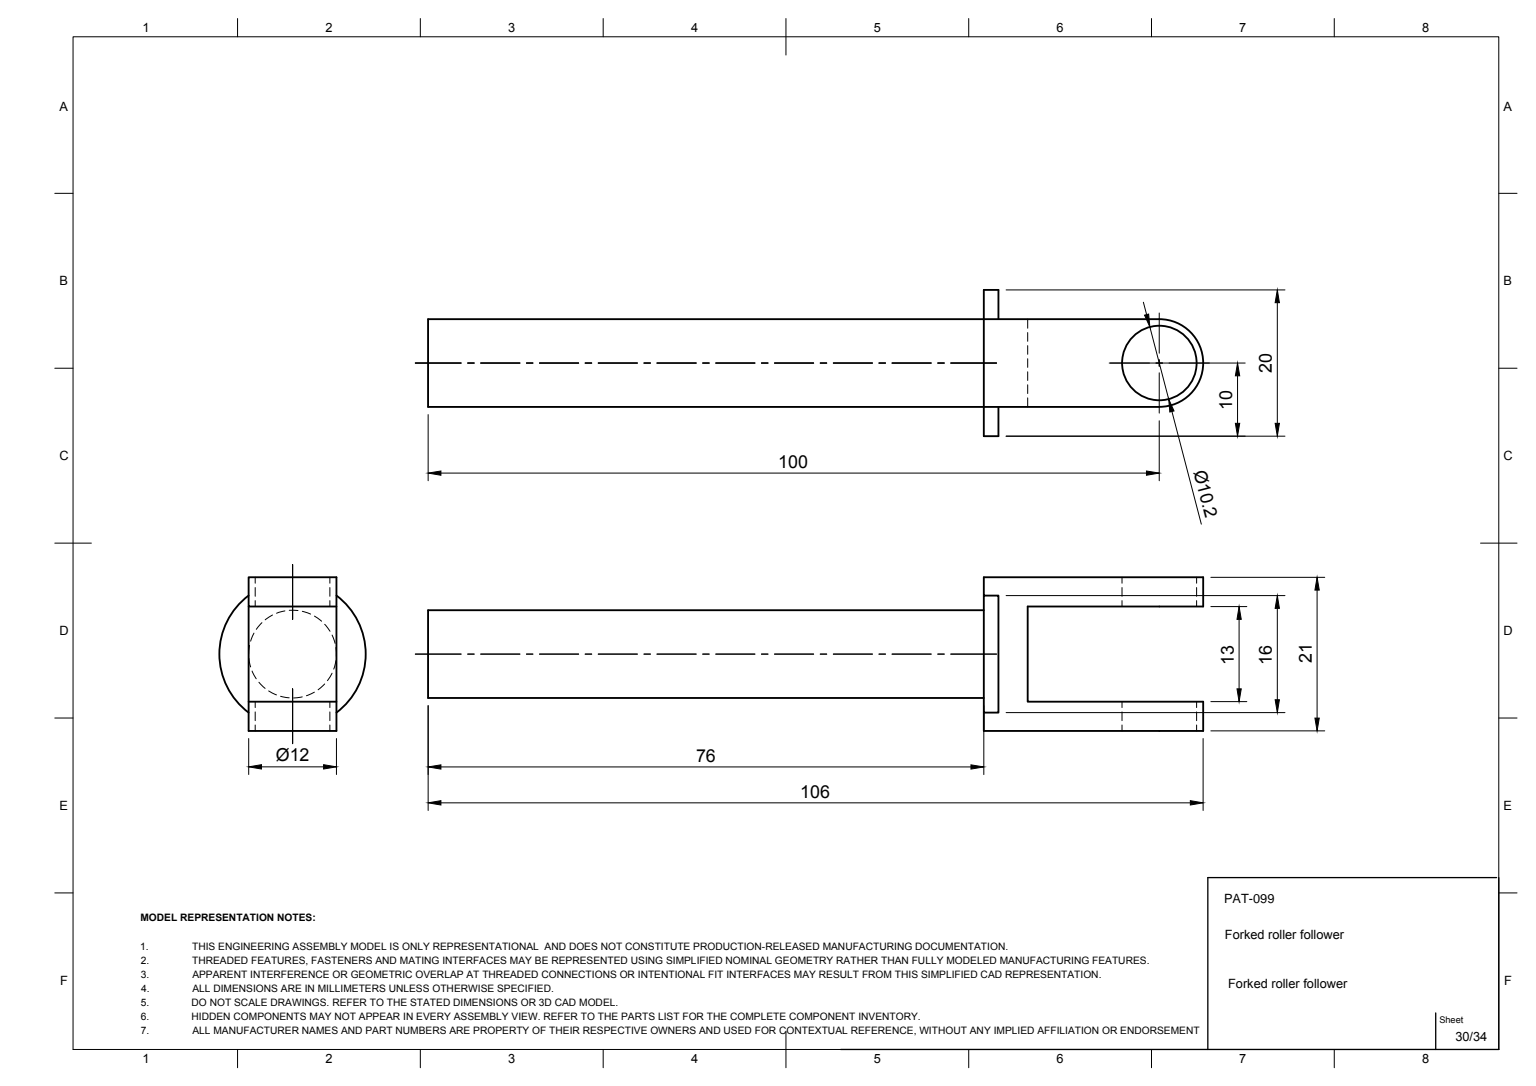
ISO-10303-21;
HEADER;
/* Generated by software containing ST-Developer
 * from STEP Tools, Inc. (www.steptools.com) 
 */

FILE_DESCRIPTION(
/* description */ ('PAT-099'),
/* implementation_level */ '2;1');

FILE_NAME(
/* name */ 'Forked roller follower.step',
/* time_stamp */ '2026-10-29T17:25:42-07:00',
/* author */ (''),
/* organization */ (''),
/* preprocessor_version */ 'ST-DEVELOPER v20.2',
/* originating_system */ 'Autodesk Translation Framework v15.17.0.0',
/* authorisation */ '');

FILE_SCHEMA (('AUTOMOTIVE_DESIGN { 1 0 10303 214 3 1 1 }'));
ENDSEC;

DATA;
#10=MECHANICAL_DESIGN_GEOMETRIC_PRESENTATION_REPRESENTATION('',(#351),#11035);
#301=SHAPE_REPRESENTATION_RELATIONSHIP('SRR','None',#11172,#326);
#326=ADVANCED_BREP_SHAPE_REPRESENTATION('',(#383),#11022);
#351=STYLED_ITEM('',(#11400),#383);
#383=MANIFOLD_SOLID_BREP('Body1',#4720);
#500=FACE_BOUND('',#1221,.T.);
#501=FACE_BOUND('',#1227,.T.);
#502=FACE_BOUND('',#1229,.T.);
#503=FACE_BOUND('',#1233,.T.);
#504=FACE_BOUND('',#1235,.T.);
#610=PLANE('',#5398);
#611=PLANE('',#5400);
#612=PLANE('',#5406);
#613=PLANE('',#5408);
#614=PLANE('',#5418);
#615=PLANE('',#5419);
#616=PLANE('',#5420);
#617=PLANE('',#5424);
#618=PLANE('',#5425);
#619=PLANE('',#5428);
#620=PLANE('',#5429);
#836=FACE_OUTER_BOUND('',#1216,.T.);
#837=FACE_OUTER_BOUND('',#1217,.T.);
#838=FACE_OUTER_BOUND('',#1218,.T.);
#839=FACE_OUTER_BOUND('',#1219,.T.);
#840=FACE_OUTER_BOUND('',#1220,.T.);
#841=FACE_OUTER_BOUND('',#1222,.T.);
#842=FACE_OUTER_BOUND('',#1223,.T.);
#843=FACE_OUTER_BOUND('',#1224,.T.);
#844=FACE_OUTER_BOUND('',#1225,.T.);
#845=FACE_OUTER_BOUND('',#1226,.T.);
#846=FACE_OUTER_BOUND('',#1228,.T.);
#847=FACE_OUTER_BOUND('',#1230,.T.);
#848=FACE_OUTER_BOUND('',#1231,.T.);
#849=FACE_OUTER_BOUND('',#1232,.T.);
#850=FACE_OUTER_BOUND('',#1234,.T.);
#851=FACE_OUTER_BOUND('',#1236,.T.);
#852=FACE_OUTER_BOUND('',#1237,.T.);
#853=FACE_OUTER_BOUND('',#1238,.T.);
#1216=EDGE_LOOP('',(#3893,#3894));
#1217=EDGE_LOOP('',(#3895,#3896));
#1218=EDGE_LOOP('',(#3897,#3898,#3899,#3900));
#1219=EDGE_LOOP('',(#3901,#3902,#3903,#3904));
#1220=EDGE_LOOP('',(#3905,#3906,#3907,#3908,#3909,#3910,#3911,#3912));
#1221=EDGE_LOOP('',(#3913));
#1222=EDGE_LOOP('',(#3914,#3915,#3916,#3917,#3918,#3919,#3920,#3921,#3922,
#3923,#3924,#3925));
#1223=EDGE_LOOP('',(#3926,#3927,#3928,#3929));
#1224=EDGE_LOOP('',(#3930,#3931,#3932,#3933));
#1225=EDGE_LOOP('',(#3934,#3935,#3936,#3937));
#1226=EDGE_LOOP('',(#3938,#3939,#3940,#3941));
#1227=EDGE_LOOP('',(#3942));
#1228=EDGE_LOOP('',(#3943,#3944,#3945,#3946));
#1229=EDGE_LOOP('',(#3947));
#1230=EDGE_LOOP('',(#3948,#3949,#3950,#3951,#3952,#3953,#3954,#3955,#3956,
#3957,#3958,#3959));
#1231=EDGE_LOOP('',(#3960,#3961,#3962,#3963));
#1232=EDGE_LOOP('',(#3964,#3965,#3966,#3967));
#1233=EDGE_LOOP('',(#3968));
#1234=EDGE_LOOP('',(#3969,#3970,#3971,#3972));
#1235=EDGE_LOOP('',(#3973));
#1236=EDGE_LOOP('',(#3974,#3975,#3976,#3977));
#1237=EDGE_LOOP('',(#3978));
#1238=EDGE_LOOP('',(#3979,#3980,#3981,#3982));
#1516=LINE('',#10121,#1768);
#1517=LINE('',#10126,#1769);
#1518=LINE('',#10130,#1770);
#1519=LINE('',#10133,#1771);
#1520=LINE('',#10136,#1772);
#1521=LINE('',#10138,#1773);
#1522=LINE('',#10142,#1774);
#1523=LINE('',#10144,#1775);
#1524=LINE('',#10145,#1776);
#1525=LINE('',#10147,#1777);
#1526=LINE('',#10149,#1778);
#1527=LINE('',#10150,#1779);
#1528=LINE('',#10155,#1780);
#1529=LINE('',#10157,#1781);
#1530=LINE('',#10159,#1782);
#1531=LINE('',#10161,#1783);
#1532=LINE('',#10163,#1784);
#1533=LINE('',#10165,#1785);
#1534=LINE('',#10166,#1786);
#1535=LINE('',#10171,#1787);
#1536=LINE('',#10177,#1788);
#1537=LINE('',#10182,#1789);
#1538=LINE('',#10186,#1790);
#1539=LINE('',#10189,#1791);
#1540=LINE('',#10190,#1792);
#1541=LINE('',#10193,#1793);
#1542=LINE('',#10195,#1794);
#1543=LINE('',#10197,#1795);
#1544=LINE('',#10198,#1796);
#1545=LINE('',#10204,#1797);
#1546=LINE('',#10208,#1798);
#1768=VECTOR('',#6607,1.);
#1769=VECTOR('',#6612,1.);
#1770=VECTOR('',#6617,1.);
#1771=VECTOR('',#6620,1.);
#1772=VECTOR('',#6623,1.);
#1773=VECTOR('',#6624,1.);
#1774=VECTOR('',#6629,1.);
#1775=VECTOR('',#6630,1.);
#1776=VECTOR('',#6631,1.);
#1777=VECTOR('',#6632,1.);
#1778=VECTOR('',#6633,1.);
#1779=VECTOR('',#6634,1.);
#1780=VECTOR('',#6639,1.);
#1781=VECTOR('',#6640,1.);
#1782=VECTOR('',#6641,1.);
#1783=VECTOR('',#6642,1.);
#1784=VECTOR('',#6643,1.);
#1785=VECTOR('',#6644,1.);
#1786=VECTOR('',#6645,1.);
#1787=VECTOR('',#6650,0.51);
#1788=VECTOR('',#6657,0.51);
#1789=VECTOR('',#6662,1.);
#1790=VECTOR('',#6669,1.);
#1791=VECTOR('',#6672,1.);
#1792=VECTOR('',#6673,1.);
#1793=VECTOR('',#6676,1.);
#1794=VECTOR('',#6677,1.);
#1795=VECTOR('',#6678,1.);
#1796=VECTOR('',#6679,1.);
#1797=VECTOR('',#6690,1.);
#1798=VECTOR('',#6695,0.6);
#2027=CIRCLE('',#5399,1.);
#2028=CIRCLE('',#5401,1.);
#2029=CIRCLE('',#5403,1.);
#2030=CIRCLE('',#5405,1.);
#2031=CIRCLE('',#5407,0.6);
#2032=CIRCLE('',#5410,0.51);
#2033=CIRCLE('',#5411,0.51);
#2034=CIRCLE('',#5413,0.51);
#2035=CIRCLE('',#5414,0.51);
#2036=CIRCLE('',#5416,0.6);
#2037=CIRCLE('',#5417,0.6);
#2038=CIRCLE('',#5422,0.6);
#2039=CIRCLE('',#5423,0.6);
#2040=CIRCLE('',#5427,0.6);
#2395=VERTEX_POINT('',#10119);
#2396=VERTEX_POINT('',#10120);
#2397=VERTEX_POINT('',#10124);
#2398=VERTEX_POINT('',#10125);
#2399=VERTEX_POINT('',#10129);
#2400=VERTEX_POINT('',#10131);
#2401=VERTEX_POINT('',#10135);
#2402=VERTEX_POINT('',#10137);
#2403=VERTEX_POINT('',#10141);
#2404=VERTEX_POINT('',#10143);
#2405=VERTEX_POINT('',#10146);
#2406=VERTEX_POINT('',#10148);
#2407=VERTEX_POINT('',#10151);
#2408=VERTEX_POINT('',#10154);
#2409=VERTEX_POINT('',#10156);
#2410=VERTEX_POINT('',#10158);
#2411=VERTEX_POINT('',#10160);
#2412=VERTEX_POINT('',#10162);
#2413=VERTEX_POINT('',#10164);
#2414=VERTEX_POINT('',#10168);
#2415=VERTEX_POINT('',#10170);
#2416=VERTEX_POINT('',#10174);
#2417=VERTEX_POINT('',#10176);
#2418=VERTEX_POINT('',#10180);
#2419=VERTEX_POINT('',#10181);
#2420=VERTEX_POINT('',#10188);
#2421=VERTEX_POINT('',#10192);
#2422=VERTEX_POINT('',#10194);
#2423=VERTEX_POINT('',#10196);
#2424=VERTEX_POINT('',#10206);
#2923=EDGE_CURVE('',#2395,#2396,#1516,.T.);
#2924=EDGE_CURVE('',#2396,#2395,#2027,.T.);
#2925=EDGE_CURVE('',#2397,#2398,#1517,.T.);
#2926=EDGE_CURVE('',#2398,#2397,#2028,.T.);
#2927=EDGE_CURVE('',#2399,#2395,#1518,.T.);
#2928=EDGE_CURVE('',#2400,#2399,#2029,.T.);
#2929=EDGE_CURVE('',#2396,#2400,#1519,.T.);
#2930=EDGE_CURVE('',#2398,#2401,#1520,.T.);
#2931=EDGE_CURVE('',#2402,#2397,#1521,.T.);
#2932=EDGE_CURVE('',#2401,#2402,#2030,.T.);
#2933=EDGE_CURVE('',#2402,#2403,#1522,.T.);
#2934=EDGE_CURVE('',#2403,#2404,#1523,.T.);
#2935=EDGE_CURVE('',#2404,#2400,#1524,.T.);
#2936=EDGE_CURVE('',#2399,#2405,#1525,.T.);
#2937=EDGE_CURVE('',#2405,#2406,#1526,.T.);
#2938=EDGE_CURVE('',#2406,#2401,#1527,.T.);
#2939=EDGE_CURVE('',#2407,#2407,#2031,.T.);
#2940=EDGE_CURVE('',#2408,#2404,#1528,.T.);
#2941=EDGE_CURVE('',#2409,#2408,#1529,.T.);
#2942=EDGE_CURVE('',#2409,#2410,#1530,.T.);
#2943=EDGE_CURVE('',#2410,#2411,#1531,.T.);
#2944=EDGE_CURVE('',#2412,#2411,#1532,.T.);
#2945=EDGE_CURVE('',#2413,#2412,#1533,.T.);
#2946=EDGE_CURVE('',#2413,#2405,#1534,.T.);
#2947=EDGE_CURVE('',#2414,#2414,#2032,.T.);
#2948=EDGE_CURVE('',#2414,#2415,#1535,.T.);
#2949=EDGE_CURVE('',#2415,#2415,#2033,.T.);
#2950=EDGE_CURVE('',#2416,#2416,#2034,.T.);
#2951=EDGE_CURVE('',#2416,#2417,#1536,.T.);
#2952=EDGE_CURVE('',#2417,#2417,#2035,.T.);
#2953=EDGE_CURVE('',#2418,#2419,#1537,.T.);
#2954=EDGE_CURVE('',#2418,#2409,#2036,.T.);
#2955=EDGE_CURVE('',#2419,#2408,#2037,.T.);
#2956=EDGE_CURVE('',#2419,#2403,#1538,.T.);
#2957=EDGE_CURVE('',#2420,#2418,#1539,.T.);
#2958=EDGE_CURVE('',#2410,#2420,#1540,.T.);
#2959=EDGE_CURVE('',#2421,#2406,#1541,.T.);
#2960=EDGE_CURVE('',#2421,#2422,#1542,.T.);
#2961=EDGE_CURVE('',#2423,#2422,#1543,.T.);
#2962=EDGE_CURVE('',#2423,#2420,#1544,.T.);
#2963=EDGE_CURVE('',#2422,#2412,#2038,.T.);
#2964=EDGE_CURVE('',#2421,#2413,#2039,.T.);
#2965=EDGE_CURVE('',#2423,#2411,#1545,.T.);
#2966=EDGE_CURVE('',#2424,#2424,#2040,.T.);
#2967=EDGE_CURVE('',#2424,#2407,#1546,.T.);
#3893=ORIENTED_EDGE('',*,*,#2923,.F.);
#3894=ORIENTED_EDGE('',*,*,#2924,.F.);
#3895=ORIENTED_EDGE('',*,*,#2925,.F.);
#3896=ORIENTED_EDGE('',*,*,#2926,.F.);
#3897=ORIENTED_EDGE('',*,*,#2927,.F.);
#3898=ORIENTED_EDGE('',*,*,#2928,.F.);
#3899=ORIENTED_EDGE('',*,*,#2929,.F.);
#3900=ORIENTED_EDGE('',*,*,#2924,.T.);
#3901=ORIENTED_EDGE('',*,*,#2930,.F.);
#3902=ORIENTED_EDGE('',*,*,#2926,.T.);
#3903=ORIENTED_EDGE('',*,*,#2931,.F.);
#3904=ORIENTED_EDGE('',*,*,#2932,.F.);
#3905=ORIENTED_EDGE('',*,*,#2933,.T.);
#3906=ORIENTED_EDGE('',*,*,#2934,.T.);
#3907=ORIENTED_EDGE('',*,*,#2935,.T.);
#3908=ORIENTED_EDGE('',*,*,#2928,.T.);
#3909=ORIENTED_EDGE('',*,*,#2936,.T.);
#3910=ORIENTED_EDGE('',*,*,#2937,.T.);
#3911=ORIENTED_EDGE('',*,*,#2938,.T.);
#3912=ORIENTED_EDGE('',*,*,#2932,.T.);
#3913=ORIENTED_EDGE('',*,*,#2939,.F.);
#3914=ORIENTED_EDGE('',*,*,#2927,.T.);
#3915=ORIENTED_EDGE('',*,*,#2923,.T.);
#3916=ORIENTED_EDGE('',*,*,#2929,.T.);
#3917=ORIENTED_EDGE('',*,*,#2935,.F.);
#3918=ORIENTED_EDGE('',*,*,#2940,.F.);
#3919=ORIENTED_EDGE('',*,*,#2941,.F.);
#3920=ORIENTED_EDGE('',*,*,#2942,.T.);
#3921=ORIENTED_EDGE('',*,*,#2943,.T.);
#3922=ORIENTED_EDGE('',*,*,#2944,.F.);
#3923=ORIENTED_EDGE('',*,*,#2945,.F.);
#3924=ORIENTED_EDGE('',*,*,#2946,.T.);
#3925=ORIENTED_EDGE('',*,*,#2936,.F.);
#3926=ORIENTED_EDGE('',*,*,#2947,.F.);
#3927=ORIENTED_EDGE('',*,*,#2948,.T.);
#3928=ORIENTED_EDGE('',*,*,#2949,.F.);
#3929=ORIENTED_EDGE('',*,*,#2948,.F.);
#3930=ORIENTED_EDGE('',*,*,#2950,.F.);
#3931=ORIENTED_EDGE('',*,*,#2951,.T.);
#3932=ORIENTED_EDGE('',*,*,#2952,.F.);
#3933=ORIENTED_EDGE('',*,*,#2951,.F.);
#3934=ORIENTED_EDGE('',*,*,#2953,.F.);
#3935=ORIENTED_EDGE('',*,*,#2954,.T.);
#3936=ORIENTED_EDGE('',*,*,#2941,.T.);
#3937=ORIENTED_EDGE('',*,*,#2955,.F.);
#3938=ORIENTED_EDGE('',*,*,#2940,.T.);
#3939=ORIENTED_EDGE('',*,*,#2934,.F.);
#3940=ORIENTED_EDGE('',*,*,#2956,.F.);
#3941=ORIENTED_EDGE('',*,*,#2955,.T.);
#3942=ORIENTED_EDGE('',*,*,#2952,.T.);
#3943=ORIENTED_EDGE('',*,*,#2957,.F.);
#3944=ORIENTED_EDGE('',*,*,#2958,.F.);
#3945=ORIENTED_EDGE('',*,*,#2942,.F.);
#3946=ORIENTED_EDGE('',*,*,#2954,.F.);
#3947=ORIENTED_EDGE('',*,*,#2950,.T.);
#3948=ORIENTED_EDGE('',*,*,#2930,.T.);
#3949=ORIENTED_EDGE('',*,*,#2938,.F.);
#3950=ORIENTED_EDGE('',*,*,#2959,.F.);
#3951=ORIENTED_EDGE('',*,*,#2960,.T.);
#3952=ORIENTED_EDGE('',*,*,#2961,.F.);
#3953=ORIENTED_EDGE('',*,*,#2962,.T.);
#3954=ORIENTED_EDGE('',*,*,#2957,.T.);
#3955=ORIENTED_EDGE('',*,*,#2953,.T.);
#3956=ORIENTED_EDGE('',*,*,#2956,.T.);
#3957=ORIENTED_EDGE('',*,*,#2933,.F.);
#3958=ORIENTED_EDGE('',*,*,#2931,.T.);
#3959=ORIENTED_EDGE('',*,*,#2925,.T.);
#3960=ORIENTED_EDGE('',*,*,#2945,.T.);
#3961=ORIENTED_EDGE('',*,*,#2963,.F.);
#3962=ORIENTED_EDGE('',*,*,#2960,.F.);
#3963=ORIENTED_EDGE('',*,*,#2964,.T.);
#3964=ORIENTED_EDGE('',*,*,#2959,.T.);
#3965=ORIENTED_EDGE('',*,*,#2937,.F.);
#3966=ORIENTED_EDGE('',*,*,#2946,.F.);
#3967=ORIENTED_EDGE('',*,*,#2964,.F.);
#3968=ORIENTED_EDGE('',*,*,#2947,.T.);
#3969=ORIENTED_EDGE('',*,*,#2944,.T.);
#3970=ORIENTED_EDGE('',*,*,#2965,.F.);
#3971=ORIENTED_EDGE('',*,*,#2961,.T.);
#3972=ORIENTED_EDGE('',*,*,#2963,.T.);
#3973=ORIENTED_EDGE('',*,*,#2949,.T.);
#3974=ORIENTED_EDGE('',*,*,#2966,.F.);
#3975=ORIENTED_EDGE('',*,*,#2967,.T.);
#3976=ORIENTED_EDGE('',*,*,#2939,.T.);
#3977=ORIENTED_EDGE('',*,*,#2967,.F.);
#3978=ORIENTED_EDGE('',*,*,#2966,.T.);
#3979=ORIENTED_EDGE('',*,*,#2958,.T.);
#3980=ORIENTED_EDGE('',*,*,#2962,.F.);
#3981=ORIENTED_EDGE('',*,*,#2965,.T.);
#3982=ORIENTED_EDGE('',*,*,#2943,.F.);
#4394=CYLINDRICAL_SURFACE('',#5402,1.);
#4395=CYLINDRICAL_SURFACE('',#5404,1.);
#4396=CYLINDRICAL_SURFACE('',#5409,0.51);
#4397=CYLINDRICAL_SURFACE('',#5412,0.51);
#4398=CYLINDRICAL_SURFACE('',#5415,0.6);
#4399=CYLINDRICAL_SURFACE('',#5421,0.6);
#4400=CYLINDRICAL_SURFACE('',#5426,0.6);
#4601=ADVANCED_FACE('',(#836),#610,.F.);
#4602=ADVANCED_FACE('',(#837),#611,.F.);
#4603=ADVANCED_FACE('',(#838),#4394,.T.);
#4604=ADVANCED_FACE('',(#839),#4395,.T.);
#4605=ADVANCED_FACE('',(#840,#500),#612,.T.);
#4606=ADVANCED_FACE('',(#841),#613,.T.);
#4607=ADVANCED_FACE('',(#842),#4396,.F.);
#4608=ADVANCED_FACE('',(#843),#4397,.F.);
#4609=ADVANCED_FACE('',(#844),#4398,.T.);
#4610=ADVANCED_FACE('',(#845,#501),#614,.T.);
#4611=ADVANCED_FACE('',(#846,#502),#615,.F.);
#4612=ADVANCED_FACE('',(#847),#616,.T.);
#4613=ADVANCED_FACE('',(#848),#4399,.T.);
#4614=ADVANCED_FACE('',(#849,#503),#617,.T.);
#4615=ADVANCED_FACE('',(#850,#504),#618,.T.);
#4616=ADVANCED_FACE('',(#851),#4400,.T.);
#4617=ADVANCED_FACE('',(#852),#619,.T.);
#4618=ADVANCED_FACE('',(#853),#620,.F.);
#4720=CLOSED_SHELL('',(#4601,#4602,#4603,#4604,#4605,#4606,#4607,#4608,
#4609,#4610,#4611,#4612,#4613,#4614,#4615,#4616,#4617,#4618));
#5397=AXIS2_PLACEMENT_3D('',#10117,#6603,#6604);
#5398=AXIS2_PLACEMENT_3D('',#10118,#6605,#6606);
#5399=AXIS2_PLACEMENT_3D('',#10122,#6608,#6609);
#5400=AXIS2_PLACEMENT_3D('',#10123,#6610,#6611);
#5401=AXIS2_PLACEMENT_3D('',#10127,#6613,#6614);
#5402=AXIS2_PLACEMENT_3D('',#10128,#6615,#6616);
#5403=AXIS2_PLACEMENT_3D('',#10132,#6618,#6619);
#5404=AXIS2_PLACEMENT_3D('',#10134,#6621,#6622);
#5405=AXIS2_PLACEMENT_3D('',#10139,#6625,#6626);
#5406=AXIS2_PLACEMENT_3D('',#10140,#6627,#6628);
#5407=AXIS2_PLACEMENT_3D('',#10152,#6635,#6636);
#5408=AXIS2_PLACEMENT_3D('',#10153,#6637,#6638);
#5409=AXIS2_PLACEMENT_3D('',#10167,#6646,#6647);
#5410=AXIS2_PLACEMENT_3D('',#10169,#6648,#6649);
#5411=AXIS2_PLACEMENT_3D('',#10172,#6651,#6652);
#5412=AXIS2_PLACEMENT_3D('',#10173,#6653,#6654);
#5413=AXIS2_PLACEMENT_3D('',#10175,#6655,#6656);
#5414=AXIS2_PLACEMENT_3D('',#10178,#6658,#6659);
#5415=AXIS2_PLACEMENT_3D('',#10179,#6660,#6661);
#5416=AXIS2_PLACEMENT_3D('',#10183,#6663,#6664);
#5417=AXIS2_PLACEMENT_3D('',#10184,#6665,#6666);
#5418=AXIS2_PLACEMENT_3D('',#10185,#6667,#6668);
#5419=AXIS2_PLACEMENT_3D('',#10187,#6670,#6671);
#5420=AXIS2_PLACEMENT_3D('',#10191,#6674,#6675);
#5421=AXIS2_PLACEMENT_3D('',#10199,#6680,#6681);
#5422=AXIS2_PLACEMENT_3D('',#10200,#6682,#6683);
#5423=AXIS2_PLACEMENT_3D('',#10201,#6684,#6685);
#5424=AXIS2_PLACEMENT_3D('',#10202,#6686,#6687);
#5425=AXIS2_PLACEMENT_3D('',#10203,#6688,#6689);
#5426=AXIS2_PLACEMENT_3D('',#10205,#6691,#6692);
#5427=AXIS2_PLACEMENT_3D('',#10207,#6693,#6694);
#5428=AXIS2_PLACEMENT_3D('',#10209,#6696,#6697);
#5429=AXIS2_PLACEMENT_3D('',#10210,#6698,#6699);
#6603=DIRECTION('axis',(0.,0.,1.));
#6604=DIRECTION('refdir',(1.,0.,0.));
#6605=DIRECTION('center_axis',(1.,0.,0.));
#6606=DIRECTION('ref_axis',(0.,0.,-1.));
#6607=DIRECTION('',(0.,0.,1.));
#6608=DIRECTION('center_axis',(1.,0.,0.));
#6609=DIRECTION('ref_axis',(0.,0.,-1.));
#6610=DIRECTION('center_axis',(1.,0.,0.));
#6611=DIRECTION('ref_axis',(0.,0.,-1.));
#6612=DIRECTION('',(0.,0.,-1.));
#6613=DIRECTION('center_axis',(1.,0.,0.));
#6614=DIRECTION('ref_axis',(0.,0.,-1.));
#6615=DIRECTION('center_axis',(1.,0.,0.));
#6616=DIRECTION('ref_axis',(0.,0.,-1.));
#6617=DIRECTION('',(-1.,0.,0.));
#6618=DIRECTION('center_axis',(1.,0.,0.));
#6619=DIRECTION('ref_axis',(0.,0.,-1.));
#6620=DIRECTION('',(1.,0.,0.));
#6621=DIRECTION('center_axis',(1.,0.,0.));
#6622=DIRECTION('ref_axis',(0.,0.,-1.));
#6623=DIRECTION('',(1.,0.,0.));
#6624=DIRECTION('',(-1.,0.,0.));
#6625=DIRECTION('center_axis',(1.,0.,0.));
#6626=DIRECTION('ref_axis',(0.,0.,-1.));
#6627=DIRECTION('center_axis',(1.,0.,0.));
#6628=DIRECTION('ref_axis',(0.,0.,-1.));
#6629=DIRECTION('',(0.,0.,1.));
#6630=DIRECTION('',(0.,-1.,0.));
#6631=DIRECTION('',(0.,0.,-1.));
#6632=DIRECTION('',(0.,0.,-1.));
#6633=DIRECTION('',(0.,1.,0.));
#6634=DIRECTION('',(0.,0.,1.));
#6635=DIRECTION('center_axis',(1.,0.,0.));
#6636=DIRECTION('ref_axis',(0.,0.,-1.));
#6637=DIRECTION('center_axis',(0.,-1.,0.));
#6638=DIRECTION('ref_axis',(0.,0.,-1.));
#6639=DIRECTION('',(1.,0.,0.));
#6640=DIRECTION('',(0.,0.,1.));
#6641=DIRECTION('',(1.,0.,0.));
#6642=DIRECTION('',(0.,0.,-1.));
#6643=DIRECTION('',(1.,0.,0.));
#6644=DIRECTION('',(0.,0.,1.));
#6645=DIRECTION('',(1.,0.,0.));
#6646=DIRECTION('center_axis',(0.,0.,1.));
#6647=DIRECTION('ref_axis',(1.,0.,0.));
#6648=DIRECTION('center_axis',(0.,0.,1.));
#6649=DIRECTION('ref_axis',(1.,0.,0.));
#6650=DIRECTION('',(0.,0.,1.));
#6651=DIRECTION('center_axis',(0.,0.,-1.));
#6652=DIRECTION('ref_axis',(1.,0.,0.));
#6653=DIRECTION('center_axis',(0.,0.,1.));
#6654=DIRECTION('ref_axis',(1.,0.,0.));
#6655=DIRECTION('center_axis',(0.,0.,1.));
#6656=DIRECTION('ref_axis',(1.,0.,0.));
#6657=DIRECTION('',(0.,0.,1.));
#6658=DIRECTION('center_axis',(0.,0.,-1.));
#6659=DIRECTION('ref_axis',(1.,0.,0.));
#6660=DIRECTION('center_axis',(0.,0.,1.));
#6661=DIRECTION('ref_axis',(-1.,1.22464679914735E-16,0.));
#6662=DIRECTION('',(0.,0.,1.));
#6663=DIRECTION('center_axis',(0.,0.,1.));
#6664=DIRECTION('ref_axis',(1.,0.,0.));
#6665=DIRECTION('center_axis',(0.,0.,1.));
#6666=DIRECTION('ref_axis',(1.,0.,0.));
#6667=DIRECTION('center_axis',(0.,0.,1.));
#6668=DIRECTION('ref_axis',(0.,-1.,0.));
#6669=DIRECTION('',(1.,0.,0.));
#6670=DIRECTION('center_axis',(0.,0.,1.));
#6671=DIRECTION('ref_axis',(1.,0.,0.));
#6672=DIRECTION('',(-1.,0.,0.));
#6673=DIRECTION('',(0.,1.,0.));
#6674=DIRECTION('center_axis',(0.,1.,0.));
#6675=DIRECTION('ref_axis',(0.,0.,1.));
#6676=DIRECTION('',(1.,0.,0.));
#6677=DIRECTION('',(0.,0.,1.));
#6678=DIRECTION('',(-1.,0.,0.));
#6679=DIRECTION('',(0.,0.,1.));
#6680=DIRECTION('center_axis',(0.,0.,1.));
#6681=DIRECTION('ref_axis',(-1.,-1.22464679914735E-16,0.));
#6682=DIRECTION('center_axis',(0.,0.,1.));
#6683=DIRECTION('ref_axis',(1.,0.,0.));
#6684=DIRECTION('center_axis',(0.,0.,1.));
#6685=DIRECTION('ref_axis',(1.,0.,0.));
#6686=DIRECTION('center_axis',(0.,0.,-1.));
#6687=DIRECTION('ref_axis',(0.,1.,0.));
#6688=DIRECTION('center_axis',(0.,0.,1.));
#6689=DIRECTION('ref_axis',(1.,0.,0.));
#6690=DIRECTION('',(0.,-1.,0.));
#6691=DIRECTION('center_axis',(1.,0.,0.));
#6692=DIRECTION('ref_axis',(0.,0.,-1.));
#6693=DIRECTION('center_axis',(1.,0.,0.));
#6694=DIRECTION('ref_axis',(0.,0.,-1.));
#6695=DIRECTION('',(-1.,0.,0.));
#6696=DIRECTION('center_axis',(1.,0.,0.));
#6697=DIRECTION('ref_axis',(0.,0.,-1.));
#6698=DIRECTION('center_axis',(1.,0.,0.));
#6699=DIRECTION('ref_axis',(0.,0.,-1.));
#10117=CARTESIAN_POINT('',(0.,0.,0.));
#10118=CARTESIAN_POINT('Origin',(6.2,0.,5.25));
#10119=CARTESIAN_POINT('',(6.2,-0.6,4.45));
#10120=CARTESIAN_POINT('',(6.2,-0.6,6.05));
#10121=CARTESIAN_POINT('',(6.2,-0.6,5.775));
#10122=CARTESIAN_POINT('Origin',(6.2,0.,5.25));
#10123=CARTESIAN_POINT('Origin',(6.2,0.,5.25));
#10124=CARTESIAN_POINT('',(6.2,0.6,6.05));
#10125=CARTESIAN_POINT('',(6.2,0.6,4.45));
#10126=CARTESIAN_POINT('',(6.2,0.6,4.725));
#10127=CARTESIAN_POINT('Origin',(6.2,0.,5.25));
#10128=CARTESIAN_POINT('Origin',(6.2,0.,5.25));
#10129=CARTESIAN_POINT('',(6.4,-0.6,4.45));
#10130=CARTESIAN_POINT('',(6.2,-0.6,4.45));
#10131=CARTESIAN_POINT('',(6.4,-0.6,6.05));
#10132=CARTESIAN_POINT('Origin',(6.4,0.,5.25));
#10133=CARTESIAN_POINT('',(6.2,-0.6,6.05));
#10134=CARTESIAN_POINT('Origin',(6.2,0.,5.25));
#10135=CARTESIAN_POINT('',(6.4,0.6,4.45));
#10136=CARTESIAN_POINT('',(6.2,0.6,4.45));
#10137=CARTESIAN_POINT('',(6.4,0.6,6.05));
#10138=CARTESIAN_POINT('',(6.2,0.6,6.05));
#10139=CARTESIAN_POINT('Origin',(6.4,0.,5.25));
#10140=CARTESIAN_POINT('Origin',(6.4,0.,5.25));
#10141=CARTESIAN_POINT('',(6.4,0.6,6.3));
#10142=CARTESIAN_POINT('',(6.4,0.6,4.2));
#10143=CARTESIAN_POINT('',(6.4,-0.6,6.3));
#10144=CARTESIAN_POINT('',(6.4,0.6,6.3));
#10145=CARTESIAN_POINT('',(6.4,-0.6,6.3));
#10146=CARTESIAN_POINT('',(6.4,-0.6,4.2));
#10147=CARTESIAN_POINT('',(6.4,-0.6,6.3));
#10148=CARTESIAN_POINT('',(6.4,0.6,4.2));
#10149=CARTESIAN_POINT('',(6.4,-0.6,4.2));
#10150=CARTESIAN_POINT('',(6.4,0.6,4.2));
#10151=CARTESIAN_POINT('',(6.4,-7.34788079488412E-17,5.85));
#10152=CARTESIAN_POINT('Origin',(6.4,0.,5.25));
#10153=CARTESIAN_POINT('Origin',(5.8,-0.6,6.3));
#10154=CARTESIAN_POINT('',(4.,-0.6,6.3));
#10155=CARTESIAN_POINT('',(4.,-0.6,6.3));
#10156=CARTESIAN_POINT('',(4.,-0.6,5.9));
#10157=CARTESIAN_POINT('',(4.,-0.6,5.9));
#10158=CARTESIAN_POINT('',(5.8,-0.6,5.9));
#10159=CARTESIAN_POINT('',(4.,-0.6,5.9));
#10160=CARTESIAN_POINT('',(5.8,-0.6,4.6));
#10161=CARTESIAN_POINT('',(5.8,-0.6,6.3));
#10162=CARTESIAN_POINT('',(4.,-0.6,4.6));
#10163=CARTESIAN_POINT('',(4.,-0.6,4.6));
#10164=CARTESIAN_POINT('',(4.,-0.6,4.2));
#10165=CARTESIAN_POINT('',(4.,-0.6,4.2));
#10166=CARTESIAN_POINT('',(5.8,-0.6,4.2));
#10167=CARTESIAN_POINT('Origin',(4.,0.,4.1));
#10168=CARTESIAN_POINT('',(3.49,-6.2456986756515E-17,4.2));
#10169=CARTESIAN_POINT('Origin',(4.,0.,4.2));
#10170=CARTESIAN_POINT('',(3.49,6.2456986756515E-17,4.6));
#10171=CARTESIAN_POINT('',(3.49,-6.2456986756515E-17,4.1));
#10172=CARTESIAN_POINT('Origin',(4.,0.,4.6));
#10173=CARTESIAN_POINT('Origin',(4.,0.,4.1));
#10174=CARTESIAN_POINT('',(3.49,-6.2456986756515E-17,5.9));
#10175=CARTESIAN_POINT('Origin',(4.,0.,5.9));
#10176=CARTESIAN_POINT('',(3.49,6.2456986756515E-17,6.3));
#10177=CARTESIAN_POINT('',(3.49,-6.2456986756515E-17,4.1));
#10178=CARTESIAN_POINT('Origin',(4.,0.,6.3));
#10179=CARTESIAN_POINT('Origin',(4.,0.,5.9));
#10180=CARTESIAN_POINT('',(4.,0.6,5.9));
#10181=CARTESIAN_POINT('',(4.,0.6,6.3));
#10182=CARTESIAN_POINT('',(4.,0.6,5.9));
#10183=CARTESIAN_POINT('Origin',(4.,0.,5.9));
#10184=CARTESIAN_POINT('Origin',(4.,0.,6.3));
#10185=CARTESIAN_POINT('Origin',(5.8,0.6,6.3));
#10186=CARTESIAN_POINT('',(5.8,0.6,6.3));
#10187=CARTESIAN_POINT('Origin',(5.05,0.,5.9));
#10188=CARTESIAN_POINT('',(5.8,0.6,5.9));
#10189=CARTESIAN_POINT('',(6.1,0.6,5.9));
#10190=CARTESIAN_POINT('',(5.8,0.,5.9));
#10191=CARTESIAN_POINT('Origin',(5.8,0.6,4.2));
#10192=CARTESIAN_POINT('',(4.,0.6,4.2));
#10193=CARTESIAN_POINT('',(5.8,0.6,4.2));
#10194=CARTESIAN_POINT('',(4.,0.6,4.6));
#10195=CARTESIAN_POINT('',(4.,0.6,4.2));
#10196=CARTESIAN_POINT('',(5.8,0.6,4.6));
#10197=CARTESIAN_POINT('',(6.1,0.6,4.6));
#10198=CARTESIAN_POINT('',(5.8,0.6,4.2));
#10199=CARTESIAN_POINT('Origin',(4.,0.,4.2));
#10200=CARTESIAN_POINT('Origin',(4.,0.,4.6));
#10201=CARTESIAN_POINT('Origin',(4.,0.,4.2));
#10202=CARTESIAN_POINT('Origin',(5.8,-0.6,4.2));
#10203=CARTESIAN_POINT('Origin',(5.05,0.,4.6));
#10204=CARTESIAN_POINT('',(5.8,0.,4.6));
#10205=CARTESIAN_POINT('Origin',(5.8,0.,5.25));
#10206=CARTESIAN_POINT('',(14.,-7.34788079488412E-17,5.85));
#10207=CARTESIAN_POINT('Origin',(14.,0.,5.25));
#10208=CARTESIAN_POINT('',(5.8,-7.34788079488412E-17,5.85));
#10209=CARTESIAN_POINT('Origin',(14.,0.,5.25));
#10210=CARTESIAN_POINT('Origin',(5.8,0.,5.25));
#10989=UNCERTAINTY_MEASURE_WITH_UNIT(LENGTH_MEASURE(0.001),#11036,
'DISTANCE_ACCURACY_VALUE',
'Maximum model space distance between geometric entities at asserted c
onnectivities');
#11002=UNCERTAINTY_MEASURE_WITH_UNIT(LENGTH_MEASURE(0.001),#11036,
'DISTANCE_ACCURACY_VALUE',
'Maximum model space distance between geometric entities at asserted c
onnectivities');
#11022=(
GEOMETRIC_REPRESENTATION_CONTEXT(3)
GLOBAL_UNCERTAINTY_ASSIGNED_CONTEXT((#10989))
GLOBAL_UNIT_ASSIGNED_CONTEXT((#11036,#11038,#11039))
REPRESENTATION_CONTEXT('','3D')
);
#11035=(
GEOMETRIC_REPRESENTATION_CONTEXT(3)
GLOBAL_UNCERTAINTY_ASSIGNED_CONTEXT((#11002))
GLOBAL_UNIT_ASSIGNED_CONTEXT((#11036,#11038,#11039))
REPRESENTATION_CONTEXT('','3D')
);
#11036=(
LENGTH_UNIT()
NAMED_UNIT(*)
SI_UNIT(.CENTI.,.METRE.)
);
#11038=(
NAMED_UNIT(*)
PLANE_ANGLE_UNIT()
SI_UNIT($,.RADIAN.)
);
#11039=(
NAMED_UNIT(*)
SI_UNIT($,.STERADIAN.)
SOLID_ANGLE_UNIT()
);
#11059=SHAPE_DEFINITION_REPRESENTATION(#11097,#11172);
#11097=PRODUCT_DEFINITION_SHAPE('',$,#11205);
#11172=SHAPE_REPRESENTATION('',(#5397),#11022);
#11185=PRODUCT_DEFINITION_CONTEXT('part definition',#11283,'design');
#11205=PRODUCT_DEFINITION('Forked roller follower',
'Forked roller follower',#11237,#11185);
#11237=PRODUCT_DEFINITION_FORMATION('',$,#11304);
#11283=APPLICATION_CONTEXT(
'Core Data for Automotive Mechanical Design Process');
#11284=PRODUCT_CONTEXT('part definition',#11283,'mechanical');
#11304=PRODUCT('Forked roller follower','Forked roller follower',
'Forked roller follower',(#11284));
#11394=COLOUR_RGB('Off White',0.89,0.88,0.83);
#11395=FILL_AREA_STYLE_COLOUR('',#11394);
#11396=FILL_AREA_STYLE('',(#11395));
#11397=SURFACE_STYLE_FILL_AREA(#11396);
#11398=SURFACE_SIDE_STYLE('',(#11397));
#11399=SURFACE_STYLE_USAGE(.BOTH.,#11398);
#11400=PRESENTATION_STYLE_ASSIGNMENT((#11399));
ENDSEC;
END-ISO-10303-21;
